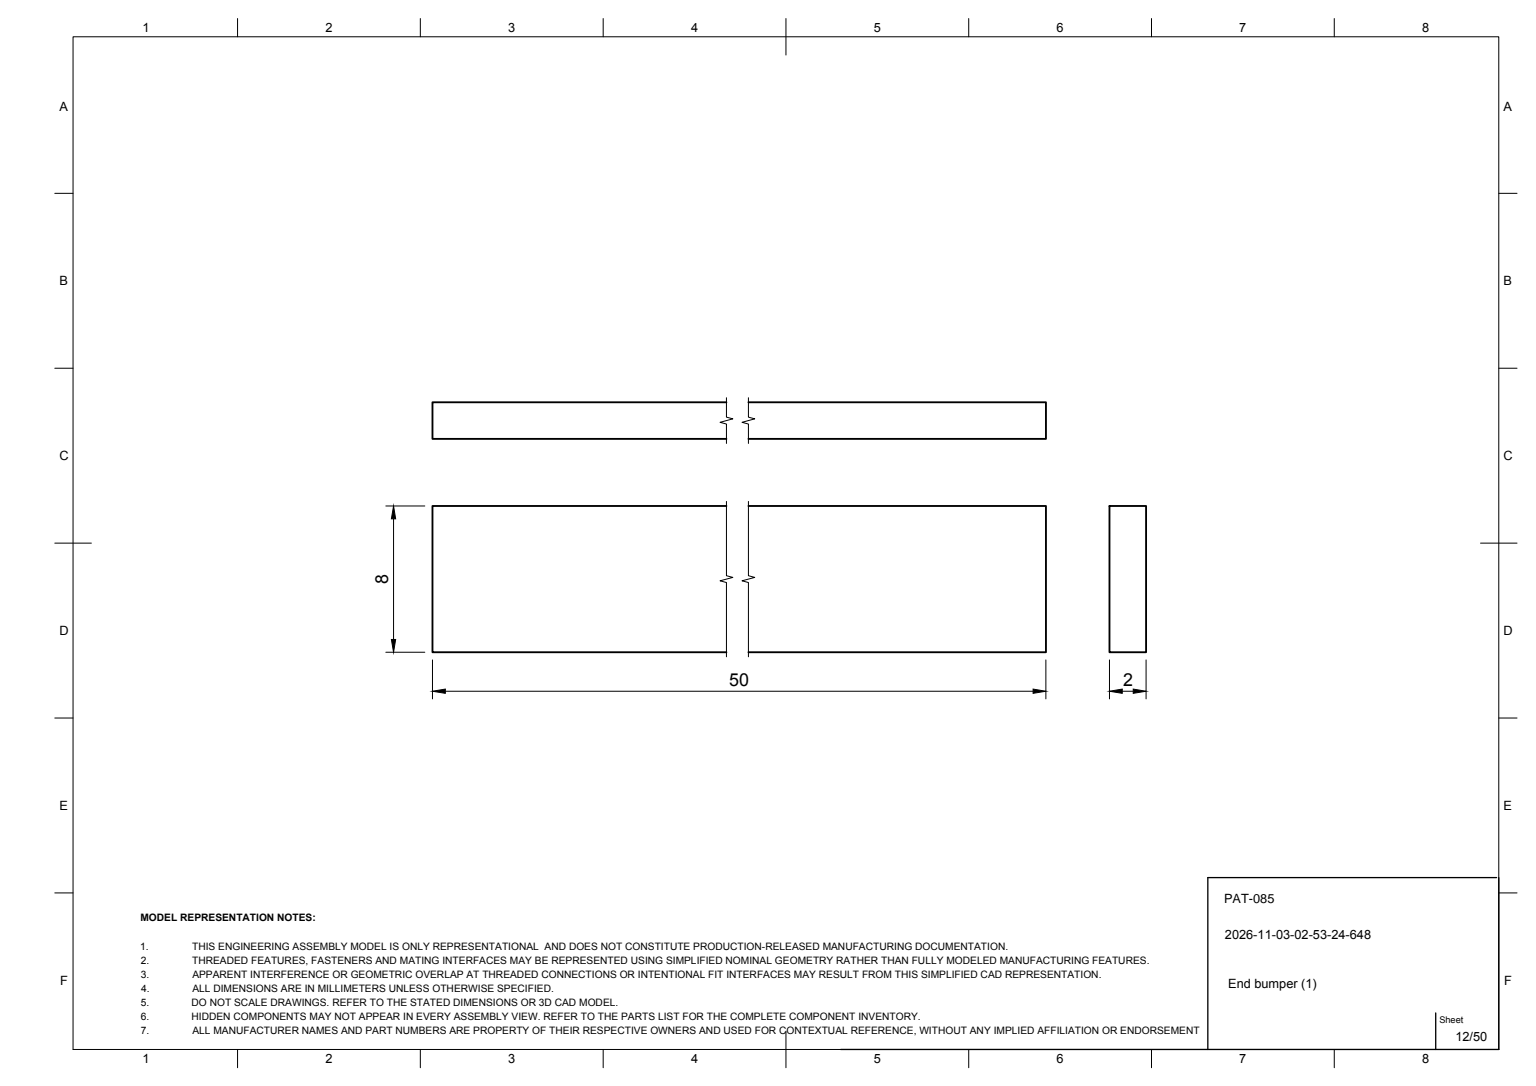
ISO-10303-21;
HEADER;
/* Generated by software containing ST-Developer
 * from STEP Tools, Inc. (www.steptools.com) 
 */

FILE_DESCRIPTION(
/* description */ ('Rack and pinion manual slide'),
/* implementation_level */ '2;1');

FILE_NAME(
/* name */ 'End bumper (1).step',
/* time_stamp */ '2026-10-28T03:22:49-07:00',
/* author */ (''),
/* organization */ (''),
/* preprocessor_version */ 'ST-DEVELOPER v20.2',
/* originating_system */ 'Autodesk Translation Framework v15.17.0.0',
/* authorisation */ '');

FILE_SCHEMA (('AUTOMOTIVE_DESIGN { 1 0 10303 214 3 1 1 }'));
ENDSEC;

DATA;
#10=MECHANICAL_DESIGN_GEOMETRIC_PRESENTATION_REPRESENTATION('',(#739),#34851);
#647=SHAPE_REPRESENTATION_RELATIONSHIP('SRR','None',#35082,#693);
#693=ADVANCED_BREP_SHAPE_REPRESENTATION('',(#792),#34807);
#739=STYLED_ITEM('',(#35404),#792);
#792=MANIFOLD_SOLID_BREP('Body1',#13759);
#1090=PLANE('',#14457);
#1091=PLANE('',#14458);
#1092=PLANE('',#14459);
#1093=PLANE('',#14460);
#1094=PLANE('',#14461);
#1095=PLANE('',#14462);
#1609=FACE_OUTER_BOUND('',#2400,.T.);
#1610=FACE_OUTER_BOUND('',#2401,.T.);
#1611=FACE_OUTER_BOUND('',#2402,.T.);
#1612=FACE_OUTER_BOUND('',#2403,.T.);
#1613=FACE_OUTER_BOUND('',#2404,.T.);
#1614=FACE_OUTER_BOUND('',#2405,.T.);
#2400=EDGE_LOOP('',(#9570,#9571,#9572,#9573));
#2401=EDGE_LOOP('',(#9574,#9575,#9576,#9577));
#2402=EDGE_LOOP('',(#9578,#9579,#9580,#9581));
#2403=EDGE_LOOP('',(#9582,#9583,#9584,#9585));
#2404=EDGE_LOOP('',(#9586,#9587,#9588,#9589));
#2405=EDGE_LOOP('',(#9590,#9591,#9592,#9593));
#3336=LINE('',#19824,#4627);
#3337=LINE('',#19826,#4628);
#3338=LINE('',#19828,#4629);
#3339=LINE('',#19829,#4630);
#3340=LINE('',#19832,#4631);
#3341=LINE('',#19834,#4632);
#3342=LINE('',#19835,#4633);
#3343=LINE('',#19838,#4634);
#3344=LINE('',#19840,#4635);
#3345=LINE('',#19841,#4636);
#3346=LINE('',#19843,#4637);
#3347=LINE('',#19844,#4638);
#4627=VECTOR('',#15994,1.);
#4628=VECTOR('',#15995,1.);
#4629=VECTOR('',#15996,1.);
#4630=VECTOR('',#15997,1.);
#4631=VECTOR('',#16000,1.);
#4632=VECTOR('',#16001,1.);
#4633=VECTOR('',#16002,1.);
#4634=VECTOR('',#16005,1.);
#4635=VECTOR('',#16006,1.);
#4636=VECTOR('',#16007,1.);
#4637=VECTOR('',#16010,1.);
#4638=VECTOR('',#16011,1.);
#6336=VERTEX_POINT('',#19822);
#6337=VERTEX_POINT('',#19823);
#6338=VERTEX_POINT('',#19825);
#6339=VERTEX_POINT('',#19827);
#6340=VERTEX_POINT('',#19831);
#6341=VERTEX_POINT('',#19833);
#6342=VERTEX_POINT('',#19837);
#6343=VERTEX_POINT('',#19839);
#7597=EDGE_CURVE('',#6336,#6337,#3336,.T.);
#7598=EDGE_CURVE('',#6337,#6338,#3337,.T.);
#7599=EDGE_CURVE('',#6339,#6338,#3338,.T.);
#7600=EDGE_CURVE('',#6336,#6339,#3339,.T.);
#7601=EDGE_CURVE('',#6340,#6336,#3340,.T.);
#7602=EDGE_CURVE('',#6341,#6339,#3341,.T.);
#7603=EDGE_CURVE('',#6340,#6341,#3342,.T.);
#7604=EDGE_CURVE('',#6342,#6340,#3343,.T.);
#7605=EDGE_CURVE('',#6343,#6341,#3344,.T.);
#7606=EDGE_CURVE('',#6342,#6343,#3345,.T.);
#7607=EDGE_CURVE('',#6337,#6342,#3346,.T.);
#7608=EDGE_CURVE('',#6338,#6343,#3347,.T.);
#9570=ORIENTED_EDGE('',*,*,#7597,.T.);
#9571=ORIENTED_EDGE('',*,*,#7598,.T.);
#9572=ORIENTED_EDGE('',*,*,#7599,.F.);
#9573=ORIENTED_EDGE('',*,*,#7600,.F.);
#9574=ORIENTED_EDGE('',*,*,#7601,.T.);
#9575=ORIENTED_EDGE('',*,*,#7600,.T.);
#9576=ORIENTED_EDGE('',*,*,#7602,.F.);
#9577=ORIENTED_EDGE('',*,*,#7603,.F.);
#9578=ORIENTED_EDGE('',*,*,#7604,.T.);
#9579=ORIENTED_EDGE('',*,*,#7603,.T.);
#9580=ORIENTED_EDGE('',*,*,#7605,.F.);
#9581=ORIENTED_EDGE('',*,*,#7606,.F.);
#9582=ORIENTED_EDGE('',*,*,#7607,.T.);
#9583=ORIENTED_EDGE('',*,*,#7606,.T.);
#9584=ORIENTED_EDGE('',*,*,#7608,.F.);
#9585=ORIENTED_EDGE('',*,*,#7598,.F.);
#9586=ORIENTED_EDGE('',*,*,#7608,.T.);
#9587=ORIENTED_EDGE('',*,*,#7605,.T.);
#9588=ORIENTED_EDGE('',*,*,#7602,.T.);
#9589=ORIENTED_EDGE('',*,*,#7599,.T.);
#9590=ORIENTED_EDGE('',*,*,#7607,.F.);
#9591=ORIENTED_EDGE('',*,*,#7597,.F.);
#9592=ORIENTED_EDGE('',*,*,#7601,.F.);
#9593=ORIENTED_EDGE('',*,*,#7604,.F.);
#13087=ADVANCED_FACE('',(#1609),#1090,.T.);
#13088=ADVANCED_FACE('',(#1610),#1091,.T.);
#13089=ADVANCED_FACE('',(#1611),#1092,.T.);
#13090=ADVANCED_FACE('',(#1612),#1093,.T.);
#13091=ADVANCED_FACE('',(#1613),#1094,.T.);
#13092=ADVANCED_FACE('',(#1614),#1095,.F.);
#13759=CLOSED_SHELL('',(#13087,#13088,#13089,#13090,#13091,#13092));
#14456=AXIS2_PLACEMENT_3D('',#19820,#15990,#15991);
#14457=AXIS2_PLACEMENT_3D('',#19821,#15992,#15993);
#14458=AXIS2_PLACEMENT_3D('',#19830,#15998,#15999);
#14459=AXIS2_PLACEMENT_3D('',#19836,#16003,#16004);
#14460=AXIS2_PLACEMENT_3D('',#19842,#16008,#16009);
#14461=AXIS2_PLACEMENT_3D('',#19845,#16012,#16013);
#14462=AXIS2_PLACEMENT_3D('',#19846,#16014,#16015);
#15990=DIRECTION('axis',(0.,0.,1.));
#15991=DIRECTION('refdir',(1.,0.,0.));
#15992=DIRECTION('center_axis',(0.,1.,0.));
#15993=DIRECTION('ref_axis',(-1.,0.,0.));
#15994=DIRECTION('',(-1.,0.,0.));
#15995=DIRECTION('',(0.,0.,1.));
#15996=DIRECTION('',(-1.,0.,0.));
#15997=DIRECTION('',(0.,0.,1.));
#15998=DIRECTION('center_axis',(1.,0.,0.));
#15999=DIRECTION('ref_axis',(0.,1.,0.));
#16000=DIRECTION('',(0.,1.,0.));
#16001=DIRECTION('',(0.,1.,0.));
#16002=DIRECTION('',(0.,0.,1.));
#16003=DIRECTION('center_axis',(0.,-1.,0.));
#16004=DIRECTION('ref_axis',(1.,0.,0.));
#16005=DIRECTION('',(1.,0.,0.));
#16006=DIRECTION('',(1.,0.,0.));
#16007=DIRECTION('',(0.,0.,1.));
#16008=DIRECTION('center_axis',(-1.,0.,0.));
#16009=DIRECTION('ref_axis',(0.,-1.,0.));
#16010=DIRECTION('',(0.,-1.,0.));
#16011=DIRECTION('',(0.,-1.,0.));
#16012=DIRECTION('center_axis',(0.,0.,1.));
#16013=DIRECTION('ref_axis',(1.,0.,0.));
#16014=DIRECTION('center_axis',(0.,0.,1.));
#16015=DIRECTION('ref_axis',(1.,0.,0.));
#19820=CARTESIAN_POINT('',(0.,0.,0.));
#19821=CARTESIAN_POINT('Origin',(25.2,2.5,6.2));
#19822=CARTESIAN_POINT('',(25.2,2.5,6.2));
#19823=CARTESIAN_POINT('',(25.,2.5,6.2));
#19824=CARTESIAN_POINT('',(25.2,2.5,6.2));
#19825=CARTESIAN_POINT('',(25.,2.5,7.));
#19826=CARTESIAN_POINT('',(25.,2.5,6.2));
#19827=CARTESIAN_POINT('',(25.2,2.5,7.));
#19828=CARTESIAN_POINT('',(25.2,2.5,7.));
#19829=CARTESIAN_POINT('',(25.2,2.5,6.2));
#19830=CARTESIAN_POINT('Origin',(25.2,-2.5,6.2));
#19831=CARTESIAN_POINT('',(25.2,-2.5,6.2));
#19832=CARTESIAN_POINT('',(25.2,-2.5,6.2));
#19833=CARTESIAN_POINT('',(25.2,-2.5,7.));
#19834=CARTESIAN_POINT('',(25.2,-2.5,7.));
#19835=CARTESIAN_POINT('',(25.2,-2.5,6.2));
#19836=CARTESIAN_POINT('Origin',(25.,-2.5,6.2));
#19837=CARTESIAN_POINT('',(25.,-2.5,6.2));
#19838=CARTESIAN_POINT('',(25.,-2.5,6.2));
#19839=CARTESIAN_POINT('',(25.,-2.5,7.));
#19840=CARTESIAN_POINT('',(25.,-2.5,7.));
#19841=CARTESIAN_POINT('',(25.,-2.5,6.2));
#19842=CARTESIAN_POINT('Origin',(25.,2.5,6.2));
#19843=CARTESIAN_POINT('',(25.,2.5,6.2));
#19844=CARTESIAN_POINT('',(25.,2.5,7.));
#19845=CARTESIAN_POINT('Origin',(25.1,0.,7.));
#19846=CARTESIAN_POINT('Origin',(25.1,0.,6.2));
#34753=UNCERTAINTY_MEASURE_WITH_UNIT(LENGTH_MEASURE(0.001),#34852,
'DISTANCE_ACCURACY_VALUE',
'Maximum model space distance between geometric entities at asserted c
onnectivities');
#34797=UNCERTAINTY_MEASURE_WITH_UNIT(LENGTH_MEASURE(0.001),#34852,
'DISTANCE_ACCURACY_VALUE',
'Maximum model space distance between geometric entities at asserted c
onnectivities');
#34807=(
GEOMETRIC_REPRESENTATION_CONTEXT(3)
GLOBAL_UNCERTAINTY_ASSIGNED_CONTEXT((#34753))
GLOBAL_UNIT_ASSIGNED_CONTEXT((#34852,#34854,#34855))
REPRESENTATION_CONTEXT('','3D')
);
#34851=(
GEOMETRIC_REPRESENTATION_CONTEXT(3)
GLOBAL_UNCERTAINTY_ASSIGNED_CONTEXT((#34797))
GLOBAL_UNIT_ASSIGNED_CONTEXT((#34852,#34854,#34855))
REPRESENTATION_CONTEXT('','3D')
);
#34852=(
LENGTH_UNIT()
NAMED_UNIT(*)
SI_UNIT(.CENTI.,.METRE.)
);
#34854=(
NAMED_UNIT(*)
PLANE_ANGLE_UNIT()
SI_UNIT($,.RADIAN.)
);
#34855=(
NAMED_UNIT(*)
SI_UNIT($,.STERADIAN.)
SOLID_ANGLE_UNIT()
);
#34865=SHAPE_DEFINITION_REPRESENTATION(#34918,#35082);
#34918=PRODUCT_DEFINITION_SHAPE('',$,#35136);
#35082=SHAPE_REPRESENTATION('',(#14456),#34807);
#35126=PRODUCT_DEFINITION_CONTEXT('part definition',#35287,'design');
#35136=PRODUCT_DEFINITION('End bumper (1)','End bumper (1)',#35189,#35126);
#35189=PRODUCT_DEFINITION_FORMATION('',$,#35298);
#35287=APPLICATION_CONTEXT(
'Core Data for Automotive Mechanical Design Process');
#35288=PRODUCT_CONTEXT('part definition',#35287,'mechanical');
#35298=PRODUCT('End bumper (1)','End bumper (1)','End bumper (1)',(#35288));
#35398=COLOUR_RGB('Sky Blue',0.24,0.69,0.87);
#35399=FILL_AREA_STYLE_COLOUR('',#35398);
#35400=FILL_AREA_STYLE('',(#35399));
#35401=SURFACE_STYLE_FILL_AREA(#35400);
#35402=SURFACE_SIDE_STYLE('',(#35401));
#35403=SURFACE_STYLE_USAGE(.BOTH.,#35402);
#35404=PRESENTATION_STYLE_ASSIGNMENT((#35403));
ENDSEC;
END-ISO-10303-21;
